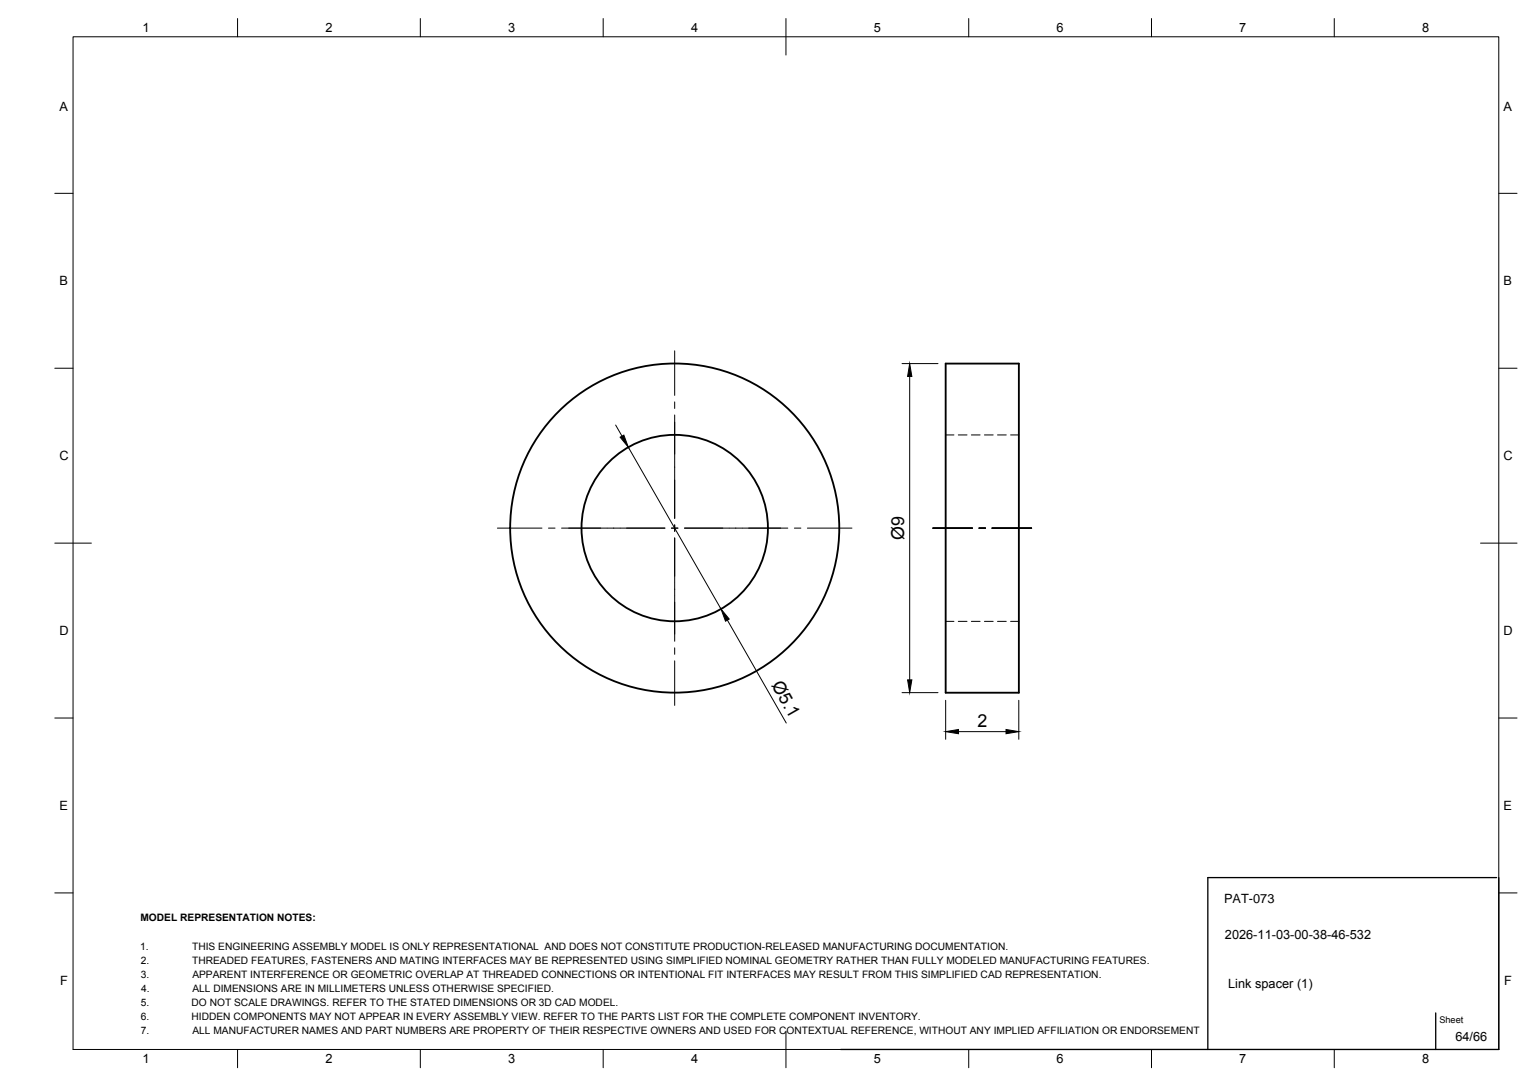
ISO-10303-21;
HEADER;
/* Generated by software containing ST-Developer
 * from STEP Tools, Inc. (www.steptools.com) 
 */

FILE_DESCRIPTION(
/* description */ ('Manual piston pump'),
/* implementation_level */ '2;1');

FILE_NAME(
/* name */ 'Link spacer (1).step',
/* time_stamp */ '2026-11-02T16:54:23-08:00',
/* author */ (''),
/* organization */ (''),
/* preprocessor_version */ 'ST-DEVELOPER v20.2',
/* originating_system */ 'Autodesk Translation Framework v15.17.0.0',
/* authorisation */ '');

FILE_SCHEMA (('AUTOMOTIVE_DESIGN { 1 0 10303 214 3 1 1 }'));
ENDSEC;

DATA;
#10=MECHANICAL_DESIGN_GEOMETRIC_PRESENTATION_REPRESENTATION('',(#756),#19043);
#621=SHAPE_REPRESENTATION_RELATIONSHIP('SRR','None',#19371,#684);
#684=ADVANCED_BREP_SHAPE_REPRESENTATION('',(#824),#19038);
#756=STYLED_ITEM('',(#19664),#824);
#824=MANIFOLD_SOLID_BREP('Body1',#9544);
#1039=FACE_BOUND('',#2625,.T.);
#1040=FACE_BOUND('',#2627,.T.);
#1282=CYLINDRICAL_SURFACE('',#11405,0.255000000000001);
#1283=CYLINDRICAL_SURFACE('',#11408,0.449999999999999);
#1835=FACE_OUTER_BOUND('',#2622,.T.);
#1836=FACE_OUTER_BOUND('',#2623,.T.);
#1837=FACE_OUTER_BOUND('',#2624,.T.);
#1838=FACE_OUTER_BOUND('',#2626,.T.);
#2622=EDGE_LOOP('',(#8453,#8454,#8455,#8456));
#2623=EDGE_LOOP('',(#8457,#8458,#8459,#8460));
#2624=EDGE_LOOP('',(#8461));
#2625=EDGE_LOOP('',(#8462));
#2626=EDGE_LOOP('',(#8463));
#2627=EDGE_LOOP('',(#8464));
#3124=CIRCLE('',#11406,0.255000000000001);
#3125=CIRCLE('',#11407,0.255000000000001);
#3126=CIRCLE('',#11409,0.449999999999999);
#3127=CIRCLE('',#11410,0.449999999999999);
#3714=LINE('',#18740,#4318);
#3715=LINE('',#18746,#4319);
#4318=VECTOR('',#14390,0.255000000000001);
#4319=VECTOR('',#14397,0.449999999999999);
#5084=VERTEX_POINT('',#18737);
#5085=VERTEX_POINT('',#18739);
#5086=VERTEX_POINT('',#18743);
#5087=VERTEX_POINT('',#18745);
#6213=EDGE_CURVE('',#5084,#5084,#3124,.T.);
#6214=EDGE_CURVE('',#5084,#5085,#3714,.T.);
#6215=EDGE_CURVE('',#5085,#5085,#3125,.T.);
#6216=EDGE_CURVE('',#5086,#5086,#3126,.T.);
#6217=EDGE_CURVE('',#5086,#5087,#3715,.T.);
#6218=EDGE_CURVE('',#5087,#5087,#3127,.T.);
#8453=ORIENTED_EDGE('',*,*,#6213,.F.);
#8454=ORIENTED_EDGE('',*,*,#6214,.T.);
#8455=ORIENTED_EDGE('',*,*,#6215,.T.);
#8456=ORIENTED_EDGE('',*,*,#6214,.F.);
#8457=ORIENTED_EDGE('',*,*,#6216,.F.);
#8458=ORIENTED_EDGE('',*,*,#6217,.T.);
#8459=ORIENTED_EDGE('',*,*,#6218,.T.);
#8460=ORIENTED_EDGE('',*,*,#6217,.F.);
#8461=ORIENTED_EDGE('',*,*,#6216,.T.);
#8462=ORIENTED_EDGE('',*,*,#6213,.T.);
#8463=ORIENTED_EDGE('',*,*,#6218,.F.);
#8464=ORIENTED_EDGE('',*,*,#6215,.F.);
#8878=PLANE('',#11411);
#8879=PLANE('',#11412);
#9440=ADVANCED_FACE('',(#1835),#1282,.F.);
#9441=ADVANCED_FACE('',(#1836),#1283,.T.);
#9442=ADVANCED_FACE('',(#1837,#1039),#8878,.T.);
#9443=ADVANCED_FACE('',(#1838,#1040),#8879,.F.);
#9544=CLOSED_SHELL('',(#9440,#9441,#9442,#9443));
#11404=AXIS2_PLACEMENT_3D('',#18735,#14384,#14385);
#11405=AXIS2_PLACEMENT_3D('',#18736,#14386,#14387);
#11406=AXIS2_PLACEMENT_3D('',#18738,#14388,#14389);
#11407=AXIS2_PLACEMENT_3D('',#18741,#14391,#14392);
#11408=AXIS2_PLACEMENT_3D('',#18742,#14393,#14394);
#11409=AXIS2_PLACEMENT_3D('',#18744,#14395,#14396);
#11410=AXIS2_PLACEMENT_3D('',#18747,#14398,#14399);
#11411=AXIS2_PLACEMENT_3D('',#18748,#14400,#14401);
#11412=AXIS2_PLACEMENT_3D('',#18749,#14402,#14403);
#14384=DIRECTION('axis',(0.,0.,1.));
#14385=DIRECTION('refdir',(1.,0.,0.));
#14386=DIRECTION('center_axis',(1.,0.,0.));
#14387=DIRECTION('ref_axis',(0.,0.,-1.));
#14388=DIRECTION('center_axis',(-1.,0.,0.));
#14389=DIRECTION('ref_axis',(0.,0.,-1.));
#14390=DIRECTION('',(-1.,0.,0.));
#14391=DIRECTION('center_axis',(-1.,0.,0.));
#14392=DIRECTION('ref_axis',(0.,0.,-1.));
#14393=DIRECTION('center_axis',(1.,0.,0.));
#14394=DIRECTION('ref_axis',(0.,0.,-1.));
#14395=DIRECTION('center_axis',(1.,0.,0.));
#14396=DIRECTION('ref_axis',(0.,0.,-1.));
#14397=DIRECTION('',(-1.,0.,0.));
#14398=DIRECTION('center_axis',(1.,0.,0.));
#14399=DIRECTION('ref_axis',(0.,0.,-1.));
#14400=DIRECTION('center_axis',(1.,0.,0.));
#14401=DIRECTION('ref_axis',(0.,0.,-1.));
#14402=DIRECTION('center_axis',(1.,0.,0.));
#14403=DIRECTION('ref_axis',(0.,0.,-1.));
#18735=CARTESIAN_POINT('',(0.,0.,0.));
#18736=CARTESIAN_POINT('Origin',(0.3,-8.,10.));
#18737=CARTESIAN_POINT('',(0.5,-8.,10.255));
#18738=CARTESIAN_POINT('Origin',(0.5,-8.,10.));
#18739=CARTESIAN_POINT('',(0.3,-8.,10.255));
#18740=CARTESIAN_POINT('',(0.3,-8.,10.255));
#18741=CARTESIAN_POINT('Origin',(0.3,-8.,10.));
#18742=CARTESIAN_POINT('Origin',(0.3,-8.,10.));
#18743=CARTESIAN_POINT('',(0.5,-8.,10.45));
#18744=CARTESIAN_POINT('Origin',(0.5,-8.,10.));
#18745=CARTESIAN_POINT('',(0.3,-8.,10.45));
#18746=CARTESIAN_POINT('',(0.3,-8.,10.45));
#18747=CARTESIAN_POINT('Origin',(0.3,-8.,10.));
#18748=CARTESIAN_POINT('Origin',(0.5,-8.,10.));
#18749=CARTESIAN_POINT('Origin',(0.3,-8.,10.));
#18967=UNCERTAINTY_MEASURE_WITH_UNIT(LENGTH_MEASURE(0.001),#19044,
'DISTANCE_ACCURACY_VALUE',
'Maximum model space distance between geometric entities at asserted c
onnectivities');
#18972=UNCERTAINTY_MEASURE_WITH_UNIT(LENGTH_MEASURE(0.001),#19044,
'DISTANCE_ACCURACY_VALUE',
'Maximum model space distance between geometric entities at asserted c
onnectivities');
#19038=(
GEOMETRIC_REPRESENTATION_CONTEXT(3)
GLOBAL_UNCERTAINTY_ASSIGNED_CONTEXT((#18967))
GLOBAL_UNIT_ASSIGNED_CONTEXT((#19044,#19046,#19047))
REPRESENTATION_CONTEXT('','3D')
);
#19043=(
GEOMETRIC_REPRESENTATION_CONTEXT(3)
GLOBAL_UNCERTAINTY_ASSIGNED_CONTEXT((#18972))
GLOBAL_UNIT_ASSIGNED_CONTEXT((#19044,#19046,#19047))
REPRESENTATION_CONTEXT('','3D')
);
#19044=(
LENGTH_UNIT()
NAMED_UNIT(*)
SI_UNIT(.CENTI.,.METRE.)
);
#19046=(
NAMED_UNIT(*)
PLANE_ANGLE_UNIT()
SI_UNIT($,.RADIAN.)
);
#19047=(
NAMED_UNIT(*)
SI_UNIT($,.STERADIAN.)
SOLID_ANGLE_UNIT()
);
#19113=SHAPE_DEFINITION_REPRESENTATION(#19270,#19371);
#19270=PRODUCT_DEFINITION_SHAPE('',$,#19442);
#19371=SHAPE_REPRESENTATION('',(#11404),#19038);
#19376=PRODUCT_DEFINITION_CONTEXT('part definition',#19588,'design');
#19442=PRODUCT_DEFINITION('2026-11-03-00-38-46-532','Link spacer (1)',#19512,
#19376);
#19512=PRODUCT_DEFINITION_FORMATION('',$,#19655);
#19588=APPLICATION_CONTEXT(
'Core Data for Automotive Mechanical Design Process');
#19589=PRODUCT_CONTEXT('part definition',#19588,'mechanical');
#19655=PRODUCT('2026-11-03-00-38-46-532','Link spacer (1)',
'Link spacer',(#19589));
#19664=PRESENTATION_STYLE_ASSIGNMENT((#19670));
#19670=SURFACE_STYLE_USAGE(.BOTH.,#19676);
#19676=SURFACE_SIDE_STYLE('',(#19682));
#19682=SURFACE_STYLE_FILL_AREA(#19688);
#19688=FILL_AREA_STYLE('CAD Library Painted - Steel gray',(#19694));
#19694=FILL_AREA_STYLE_COLOUR('CAD Library Painted - Steel gray',#19700);
#19700=COLOUR_RGB('CAD Library Painted - Steel gray',0.592156862745098,
0.631372549019608,0.67843137254902);
ENDSEC;
END-ISO-10303-21;
